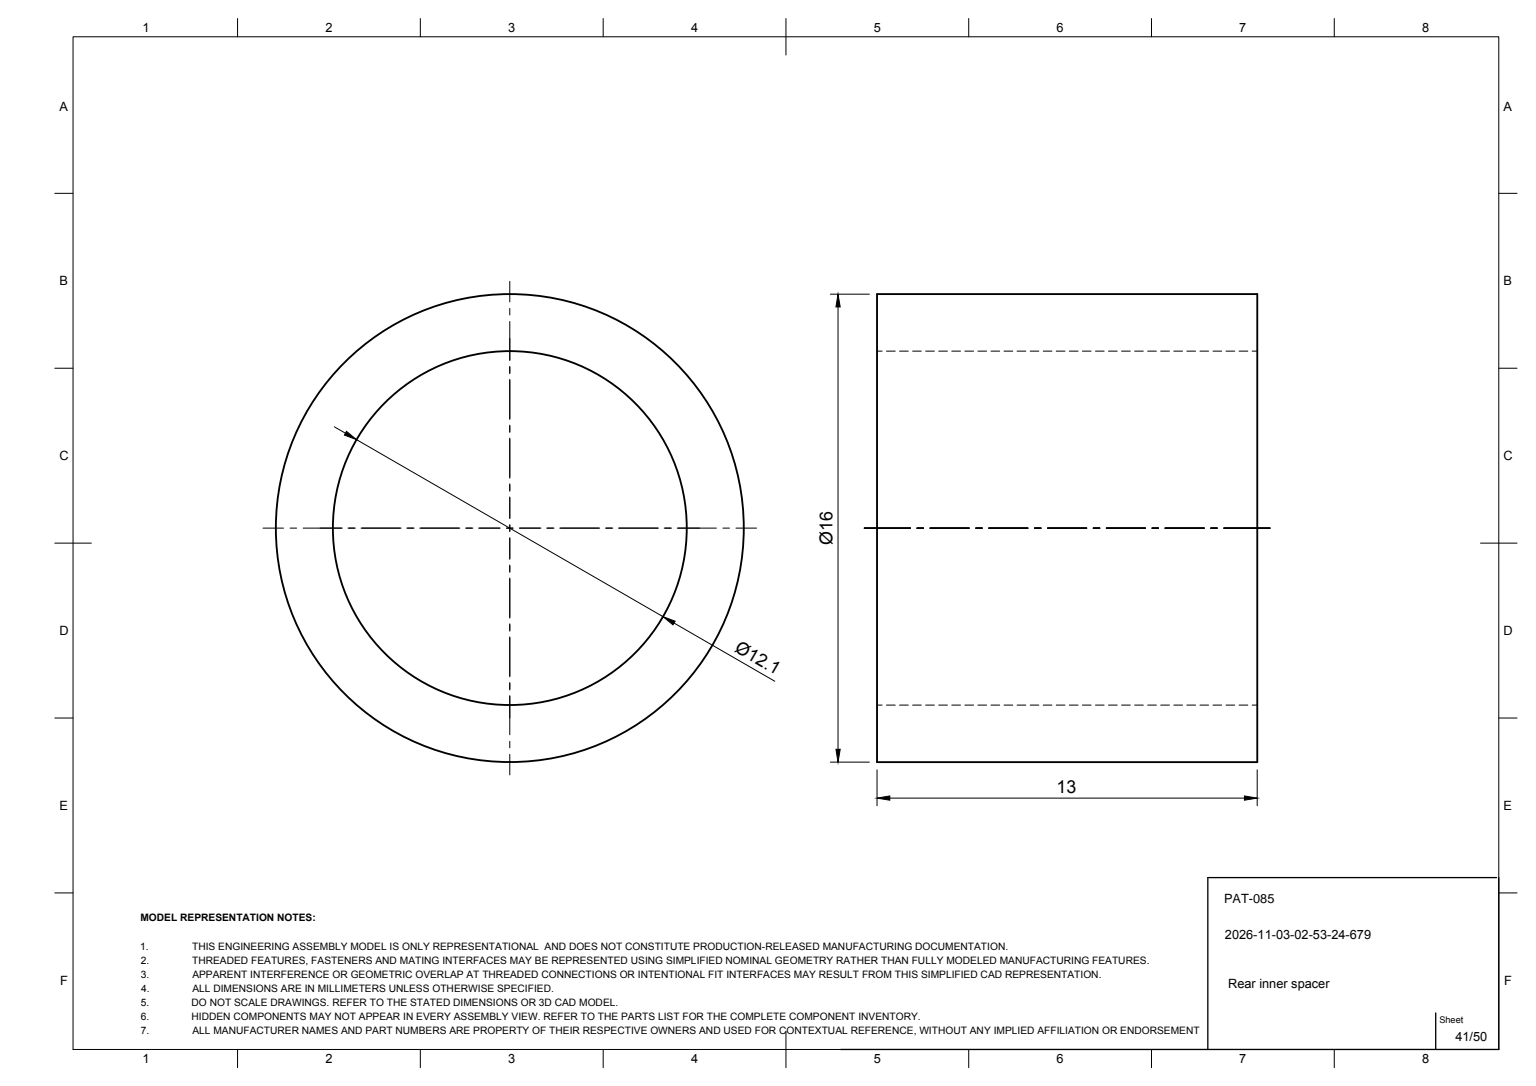
ISO-10303-21;
HEADER;
/* Generated by software containing ST-Developer
 * from STEP Tools, Inc. (www.steptools.com) 
 */

FILE_DESCRIPTION(
/* description */ ('Rack and pinion manual slide'),
/* implementation_level */ '2;1');

FILE_NAME(
/* name */ 'Rear inner spacer.step',
/* time_stamp */ '2026-10-28T03:22:49-07:00',
/* author */ (''),
/* organization */ (''),
/* preprocessor_version */ 'ST-DEVELOPER v20.2',
/* originating_system */ 'Autodesk Translation Framework v15.17.0.0',
/* authorisation */ '');

FILE_SCHEMA (('AUTOMOTIVE_DESIGN { 1 0 10303 214 3 1 1 }'));
ENDSEC;

DATA;
#10=MECHANICAL_DESIGN_GEOMETRIC_PRESENTATION_REPRESENTATION('',(#772),#34851);
#673=SHAPE_REPRESENTATION_RELATIONSHIP('SRR','None',#35112,#719);
#719=ADVANCED_BREP_SHAPE_REPRESENTATION('',(#822),#34837);
#772=STYLED_ITEM('',(#35404),#822);
#822=MANIFOLD_SOLID_BREP('Body1',#13795);
#1018=FACE_BOUND('',#3024,.T.);
#1019=FACE_BOUND('',#3026,.T.);
#1452=PLANE('',#15251);
#1453=PLANE('',#15252);
#2097=FACE_OUTER_BOUND('',#3021,.T.);
#2098=FACE_OUTER_BOUND('',#3022,.T.);
#2099=FACE_OUTER_BOUND('',#3023,.T.);
#2100=FACE_OUTER_BOUND('',#3025,.T.);
#3021=EDGE_LOOP('',(#12002,#12003,#12004,#12005));
#3022=EDGE_LOOP('',(#12006,#12007,#12008,#12009));
#3023=EDGE_LOOP('',(#12010));
#3024=EDGE_LOOP('',(#12011));
#3025=EDGE_LOOP('',(#12012));
#3026=EDGE_LOOP('',(#12013));
#4276=LINE('',#22676,#5567);
#4277=LINE('',#22682,#5568);
#5567=VECTOR('',#18512,0.605);
#5568=VECTOR('',#18519,0.800000000000001);
#6122=CIRCLE('',#15246,0.605);
#6123=CIRCLE('',#15247,0.605);
#6124=CIRCLE('',#15249,0.800000000000001);
#6125=CIRCLE('',#15250,0.800000000000001);
#7151=VERTEX_POINT('',#22673);
#7152=VERTEX_POINT('',#22675);
#7153=VERTEX_POINT('',#22679);
#7154=VERTEX_POINT('',#22681);
#8813=EDGE_CURVE('',#7151,#7151,#6122,.T.);
#8814=EDGE_CURVE('',#7151,#7152,#4276,.T.);
#8815=EDGE_CURVE('',#7152,#7152,#6123,.T.);
#8816=EDGE_CURVE('',#7153,#7153,#6124,.T.);
#8817=EDGE_CURVE('',#7153,#7154,#4277,.T.);
#8818=EDGE_CURVE('',#7154,#7154,#6125,.T.);
#12002=ORIENTED_EDGE('',*,*,#8813,.F.);
#12003=ORIENTED_EDGE('',*,*,#8814,.T.);
#12004=ORIENTED_EDGE('',*,*,#8815,.T.);
#12005=ORIENTED_EDGE('',*,*,#8814,.F.);
#12006=ORIENTED_EDGE('',*,*,#8816,.F.);
#12007=ORIENTED_EDGE('',*,*,#8817,.T.);
#12008=ORIENTED_EDGE('',*,*,#8818,.T.);
#12009=ORIENTED_EDGE('',*,*,#8817,.F.);
#12010=ORIENTED_EDGE('',*,*,#8816,.T.);
#12011=ORIENTED_EDGE('',*,*,#8813,.T.);
#12012=ORIENTED_EDGE('',*,*,#8818,.F.);
#12013=ORIENTED_EDGE('',*,*,#8815,.F.);
#12967=CYLINDRICAL_SURFACE('',#15245,0.605);
#12968=CYLINDRICAL_SURFACE('',#15248,0.800000000000001);
#13575=ADVANCED_FACE('',(#2097),#12967,.F.);
#13576=ADVANCED_FACE('',(#2098),#12968,.T.);
#13577=ADVANCED_FACE('',(#2099,#1018),#1452,.T.);
#13578=ADVANCED_FACE('',(#2100,#1019),#1453,.F.);
#13795=CLOSED_SHELL('',(#13575,#13576,#13577,#13578));
#15244=AXIS2_PLACEMENT_3D('',#22671,#18506,#18507);
#15245=AXIS2_PLACEMENT_3D('',#22672,#18508,#18509);
#15246=AXIS2_PLACEMENT_3D('',#22674,#18510,#18511);
#15247=AXIS2_PLACEMENT_3D('',#22677,#18513,#18514);
#15248=AXIS2_PLACEMENT_3D('',#22678,#18515,#18516);
#15249=AXIS2_PLACEMENT_3D('',#22680,#18517,#18518);
#15250=AXIS2_PLACEMENT_3D('',#22683,#18520,#18521);
#15251=AXIS2_PLACEMENT_3D('',#22684,#18522,#18523);
#15252=AXIS2_PLACEMENT_3D('',#22685,#18524,#18525);
#18506=DIRECTION('axis',(0.,0.,1.));
#18507=DIRECTION('refdir',(1.,0.,0.));
#18508=DIRECTION('center_axis',(0.,1.,0.));
#18509=DIRECTION('ref_axis',(1.,0.,0.));
#18510=DIRECTION('center_axis',(0.,-1.,0.));
#18511=DIRECTION('ref_axis',(1.,0.,0.));
#18512=DIRECTION('',(0.,-1.,0.));
#18513=DIRECTION('center_axis',(0.,-1.,0.));
#18514=DIRECTION('ref_axis',(1.,0.,0.));
#18515=DIRECTION('center_axis',(0.,1.,0.));
#18516=DIRECTION('ref_axis',(1.,0.,0.));
#18517=DIRECTION('center_axis',(0.,1.,0.));
#18518=DIRECTION('ref_axis',(1.,0.,0.));
#18519=DIRECTION('',(0.,-1.,0.));
#18520=DIRECTION('center_axis',(0.,1.,0.));
#18521=DIRECTION('ref_axis',(1.,0.,0.));
#18522=DIRECTION('center_axis',(0.,1.,0.));
#18523=DIRECTION('ref_axis',(1.,0.,0.));
#18524=DIRECTION('center_axis',(0.,1.,0.));
#18525=DIRECTION('ref_axis',(1.,0.,0.));
#22671=CARTESIAN_POINT('',(0.,0.,0.));
#22672=CARTESIAN_POINT('Origin',(11.,-6.,10.25));
#22673=CARTESIAN_POINT('',(10.395,-4.7,10.25));
#22674=CARTESIAN_POINT('Origin',(11.,-4.7,10.25));
#22675=CARTESIAN_POINT('',(10.395,-6.,10.25));
#22676=CARTESIAN_POINT('',(10.395,-6.,10.25));
#22677=CARTESIAN_POINT('Origin',(11.,-6.,10.25));
#22678=CARTESIAN_POINT('Origin',(11.,-6.,10.25));
#22679=CARTESIAN_POINT('',(10.2,-4.7,10.25));
#22680=CARTESIAN_POINT('Origin',(11.,-4.7,10.25));
#22681=CARTESIAN_POINT('',(10.2,-6.,10.25));
#22682=CARTESIAN_POINT('',(10.2,-6.,10.25));
#22683=CARTESIAN_POINT('Origin',(11.,-6.,10.25));
#22684=CARTESIAN_POINT('Origin',(11.,-4.7,10.25));
#22685=CARTESIAN_POINT('Origin',(11.,-6.,10.25));
#34783=UNCERTAINTY_MEASURE_WITH_UNIT(LENGTH_MEASURE(0.001),#34852,
'DISTANCE_ACCURACY_VALUE',
'Maximum model space distance between geometric entities at asserted c
onnectivities');
#34797=UNCERTAINTY_MEASURE_WITH_UNIT(LENGTH_MEASURE(0.001),#34852,
'DISTANCE_ACCURACY_VALUE',
'Maximum model space distance between geometric entities at asserted c
onnectivities');
#34837=(
GEOMETRIC_REPRESENTATION_CONTEXT(3)
GLOBAL_UNCERTAINTY_ASSIGNED_CONTEXT((#34783))
GLOBAL_UNIT_ASSIGNED_CONTEXT((#34852,#34854,#34855))
REPRESENTATION_CONTEXT('','3D')
);
#34851=(
GEOMETRIC_REPRESENTATION_CONTEXT(3)
GLOBAL_UNCERTAINTY_ASSIGNED_CONTEXT((#34797))
GLOBAL_UNIT_ASSIGNED_CONTEXT((#34852,#34854,#34855))
REPRESENTATION_CONTEXT('','3D')
);
#34852=(
LENGTH_UNIT()
NAMED_UNIT(*)
SI_UNIT(.CENTI.,.METRE.)
);
#34854=(
NAMED_UNIT(*)
PLANE_ANGLE_UNIT()
SI_UNIT($,.RADIAN.)
);
#34855=(
NAMED_UNIT(*)
SI_UNIT($,.STERADIAN.)
SOLID_ANGLE_UNIT()
);
#34895=SHAPE_DEFINITION_REPRESENTATION(#34956,#35112);
#34956=PRODUCT_DEFINITION_SHAPE('',$,#35166);
#35112=SHAPE_REPRESENTATION('',(#15244),#34837);
#35126=PRODUCT_DEFINITION_CONTEXT('part definition',#35287,'design');
#35166=PRODUCT_DEFINITION('Rear inner spacer','Rear inner spacer',#35219,
#35126);
#35219=PRODUCT_DEFINITION_FORMATION('',$,#35328);
#35287=APPLICATION_CONTEXT(
'Core Data for Automotive Mechanical Design Process');
#35288=PRODUCT_CONTEXT('part definition',#35287,'mechanical');
#35328=PRODUCT('Rear inner spacer','Rear inner spacer',
'Rear inner spacer',(#35288));
#35398=COLOUR_RGB('Sky Blue',0.24,0.69,0.87);
#35399=FILL_AREA_STYLE_COLOUR('',#35398);
#35400=FILL_AREA_STYLE('',(#35399));
#35401=SURFACE_STYLE_FILL_AREA(#35400);
#35402=SURFACE_SIDE_STYLE('',(#35401));
#35403=SURFACE_STYLE_USAGE(.BOTH.,#35402);
#35404=PRESENTATION_STYLE_ASSIGNMENT((#35403));
ENDSEC;
END-ISO-10303-21;
